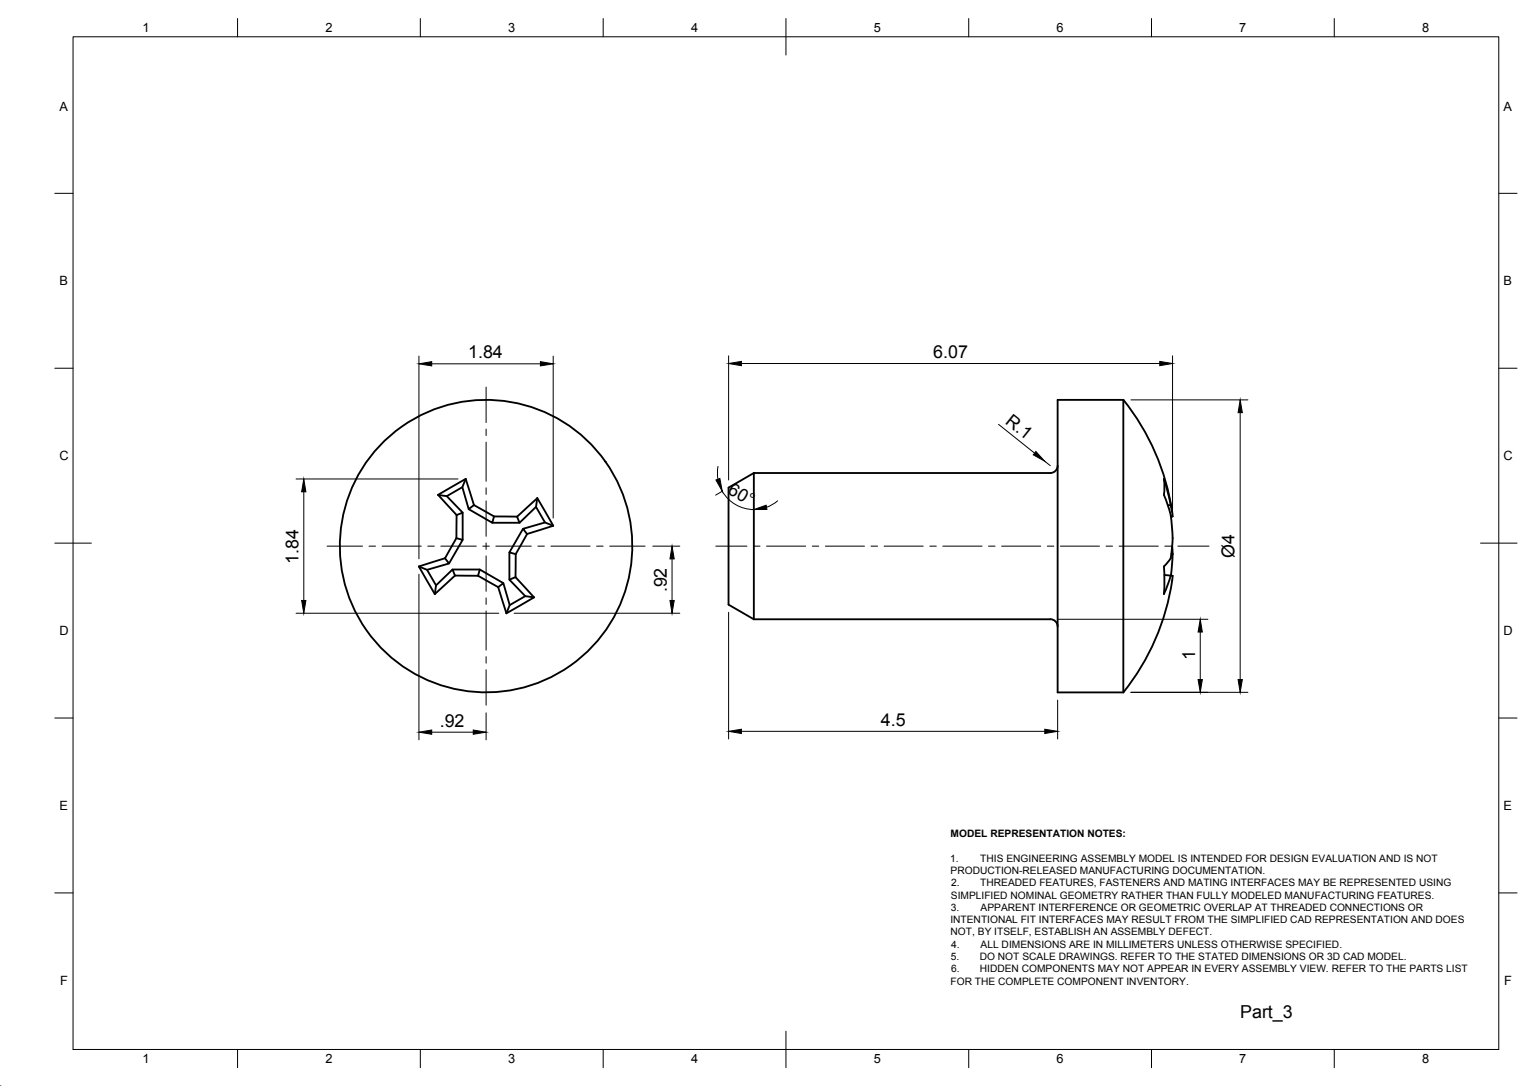
ISO-10303-21;
HEADER;
/* Generated by software containing ST-Developer
 * from STEP Tools, Inc. (www.steptools.com) 
 */

FILE_DESCRIPTION(
/* description */ ('STEP AP242 Edition 2'),
/* implementation_level */ '2;1');

FILE_NAME(
/* name */ 'Part_3.step',
/* time_stamp */ '2026-10-06T10:11:12-07:00',
/* author */ (''),
/* organization */ (''),
/* preprocessor_version */ 'ST-DEVELOPER v20.2',
/* originating_system */ 'Autodesk Translation Framework v15.15.0.0',
/* authorisation */ '');

FILE_SCHEMA (('AUTOMOTIVE_DESIGN { 1 0 10303 214 3 1 1 }'));
ENDSEC;

DATA;
#10=MECHANICAL_DESIGN_GEOMETRIC_PRESENTATION_REPRESENTATION('',(#1796),#54580);
#141=CONICAL_SURFACE('',#19114,0.001,0.5235987755983);
#151=SPHERICAL_SURFACE('',#19080,0.0032);
#260=TOROIDAL_SURFACE('',#19136,0.0011,0.0001);
#1752=SHAPE_REPRESENTATION_RELATIONSHIP('SRR','None',#54639,#1766);
#1766=ADVANCED_BREP_SHAPE_REPRESENTATION('',(#1810),#54575);
#1796=STYLED_ITEM('',(#54716),#1810);
#1810=MANIFOLD_SOLID_BREP('Body1',#17675);
#2262=LINE('',#48636,#2855);
#2263=LINE('',#48644,#2856);
#2264=LINE('',#48647,#2857);
#2265=LINE('',#48650,#2858);
#2266=LINE('',#48652,#2859);
#2267=LINE('',#48653,#2860);
#2268=LINE('',#48656,#2861);
#2269=LINE('',#48657,#2862);
#2270=LINE('',#48660,#2863);
#2271=LINE('',#48661,#2864);
#2272=LINE('',#48664,#2865);
#2273=LINE('',#48665,#2866);
#2274=LINE('',#48668,#2867);
#2275=LINE('',#48669,#2868);
#2276=LINE('',#48672,#2869);
#2277=LINE('',#48673,#2870);
#2278=LINE('',#48676,#2871);
#2279=LINE('',#48677,#2872);
#2280=LINE('',#48680,#2873);
#2281=LINE('',#48681,#2874);
#2282=LINE('',#48684,#2875);
#2283=LINE('',#48685,#2876);
#2284=LINE('',#48688,#2877);
#2285=LINE('',#48689,#2878);
#2286=LINE('',#48692,#2879);
#2287=LINE('',#48693,#2880);
#2288=LINE('',#48696,#2881);
#2289=LINE('',#48697,#2882);
#2290=LINE('',#48700,#2883);
#2291=LINE('',#48701,#2884);
#2292=LINE('',#48704,#2885);
#2293=LINE('',#48705,#2886);
#2294=LINE('',#48708,#2887);
#2295=LINE('',#48709,#2888);
#2296=LINE('',#48712,#2889);
#2297=LINE('',#48713,#2890);
#2298=LINE('',#48716,#2891);
#2299=LINE('',#48717,#2892);
#2300=LINE('',#48720,#2893);
#2301=LINE('',#48721,#2894);
#2302=LINE('',#48724,#2895);
#2303=LINE('',#48725,#2896);
#2304=LINE('',#48727,#2897);
#2855=VECTOR('',#22596,0.002);
#2856=VECTOR('',#22605,0.001);
#2857=VECTOR('',#22610,0.001);
#2858=VECTOR('',#22613,1.);
#2859=VECTOR('',#22614,1.);
#2860=VECTOR('',#22615,1.);
#2861=VECTOR('',#22618,1.);
#2862=VECTOR('',#22619,1.);
#2863=VECTOR('',#22622,1.);
#2864=VECTOR('',#22623,1.);
#2865=VECTOR('',#22626,1.);
#2866=VECTOR('',#22627,1.);
#2867=VECTOR('',#22630,1.);
#2868=VECTOR('',#22631,1.);
#2869=VECTOR('',#22634,0.999999999999999);
#2870=VECTOR('',#22635,1.);
#2871=VECTOR('',#22638,1.);
#2872=VECTOR('',#22639,1.);
#2873=VECTOR('',#22642,1.);
#2874=VECTOR('',#22643,1.);
#2875=VECTOR('',#22646,1.);
#2876=VECTOR('',#22647,1.);
#2877=VECTOR('',#22650,1.);
#2878=VECTOR('',#22651,1.);
#2879=VECTOR('',#22654,1.);
#2880=VECTOR('',#22655,1.);
#2881=VECTOR('',#22658,1.);
#2882=VECTOR('',#22659,1.);
#2883=VECTOR('',#22662,1.);
#2884=VECTOR('',#22663,1.);
#2885=VECTOR('',#22666,1.);
#2886=VECTOR('',#22667,1.);
#2887=VECTOR('',#22670,1.);
#2888=VECTOR('',#22671,1.);
#2889=VECTOR('',#22674,1.);
#2890=VECTOR('',#22675,1.);
#2891=VECTOR('',#22678,1.);
#2892=VECTOR('',#22679,0.999999999999999);
#2893=VECTOR('',#22682,1.);
#2894=VECTOR('',#22683,1.);
#2895=VECTOR('',#22686,1.);
#2896=VECTOR('',#22687,1.);
#2897=VECTOR('',#22690,1.);
#3400=CYLINDRICAL_SURFACE('',#19108,0.002);
#3401=CYLINDRICAL_SURFACE('',#19111,0.001);
#3513=FACE_BOUND('',#5345,.T.);
#4301=FACE_OUTER_BOUND('',#5343,.T.);
#4302=FACE_OUTER_BOUND('',#5344,.T.);
#4303=FACE_OUTER_BOUND('',#5346,.T.);
#4304=FACE_OUTER_BOUND('',#5347,.T.);
#4305=FACE_OUTER_BOUND('',#5348,.T.);
#4306=FACE_OUTER_BOUND('',#5349,.T.);
#4307=FACE_OUTER_BOUND('',#5350,.T.);
#4308=FACE_OUTER_BOUND('',#5351,.T.);
#4309=FACE_OUTER_BOUND('',#5352,.T.);
#4310=FACE_OUTER_BOUND('',#5353,.T.);
#4311=FACE_OUTER_BOUND('',#5354,.T.);
#4312=FACE_OUTER_BOUND('',#5355,.T.);
#4313=FACE_OUTER_BOUND('',#5356,.T.);
#4314=FACE_OUTER_BOUND('',#5357,.T.);
#4315=FACE_OUTER_BOUND('',#5358,.T.);
#4316=FACE_OUTER_BOUND('',#5359,.T.);
#4317=FACE_OUTER_BOUND('',#5360,.T.);
#4318=FACE_OUTER_BOUND('',#5361,.T.);
#4319=FACE_OUTER_BOUND('',#5362,.T.);
#4320=FACE_OUTER_BOUND('',#5363,.T.);
#4321=FACE_OUTER_BOUND('',#5364,.T.);
#4322=FACE_OUTER_BOUND('',#5365,.T.);
#4323=FACE_OUTER_BOUND('',#5366,.T.);
#4324=FACE_OUTER_BOUND('',#5367,.T.);
#4325=FACE_OUTER_BOUND('',#5368,.T.);
#4326=FACE_OUTER_BOUND('',#5369,.T.);
#4327=FACE_OUTER_BOUND('',#5370,.T.);
#4328=FACE_OUTER_BOUND('',#5371,.T.);
#5343=EDGE_LOOP('',(#15325,#15326,#15327,#15328,#15329,#15330,#15331,#15332,
#15333,#15334,#15335,#15336,#15337,#15338,#15339,#15340,#15341,#15342,#15343,
#15344,#15345,#15346,#15347,#15348,#15349));
#5344=EDGE_LOOP('',(#15350));
#5345=EDGE_LOOP('',(#15351));
#5346=EDGE_LOOP('',(#15352,#15353,#15354,#15355,#15356));
#5347=EDGE_LOOP('',(#15357));
#5348=EDGE_LOOP('',(#15358,#15359,#15360,#15361));
#5349=EDGE_LOOP('',(#15362,#15363,#15364,#15365));
#5350=EDGE_LOOP('',(#15366,#15367,#15368,#15369));
#5351=EDGE_LOOP('',(#15370,#15371,#15372,#15373));
#5352=EDGE_LOOP('',(#15374,#15375,#15376,#15377));
#5353=EDGE_LOOP('',(#15378,#15379,#15380,#15381));
#5354=EDGE_LOOP('',(#15382,#15383,#15384,#15385));
#5355=EDGE_LOOP('',(#15386,#15387,#15388,#15389));
#5356=EDGE_LOOP('',(#15390,#15391,#15392,#15393));
#5357=EDGE_LOOP('',(#15394,#15395,#15396,#15397));
#5358=EDGE_LOOP('',(#15398,#15399,#15400,#15401));
#5359=EDGE_LOOP('',(#15402,#15403,#15404,#15405));
#5360=EDGE_LOOP('',(#15406,#15407,#15408,#15409));
#5361=EDGE_LOOP('',(#15410,#15411,#15412,#15413,#15414));
#5362=EDGE_LOOP('',(#15415,#15416,#15417,#15418));
#5363=EDGE_LOOP('',(#15419,#15420,#15421,#15422));
#5364=EDGE_LOOP('',(#15423,#15424,#15425,#15426));
#5365=EDGE_LOOP('',(#15427,#15428,#15429,#15430));
#5366=EDGE_LOOP('',(#15431,#15432,#15433,#15434));
#5367=EDGE_LOOP('',(#15435,#15436,#15437,#15438));
#5368=EDGE_LOOP('',(#15439,#15440,#15441,#15442));
#5369=EDGE_LOOP('',(#15443,#15444,#15445,#15446));
#5370=EDGE_LOOP('',(#15447,#15448,#15449,#15450,#15451,#15452,#15453,#15454,
#15455,#15456,#15457,#15458,#15459,#15460,#15461,#15462,#15463,#15464,#15465,
#15466));
#5371=EDGE_LOOP('',(#15467,#15468,#15469,#15470));
#6242=CIRCLE('',#19081,0.00318247006517847);
#6243=CIRCLE('',#19082,0.00314126219074625);
#6244=CIRCLE('',#19083,0.00318247006517847);
#6245=CIRCLE('',#19084,0.00319919707806175);
#6246=CIRCLE('',#19085,0.00319919707806175);
#6247=CIRCLE('',#19086,0.00318247006517847);
#6248=CIRCLE('',#19087,0.00314126219074625);
#6249=CIRCLE('',#19088,0.00318247006517847);
#6250=CIRCLE('',#19089,0.00319919707806175);
#6251=CIRCLE('',#19090,0.00319919707806175);
#6252=CIRCLE('',#19091,0.00318247006517847);
#6253=CIRCLE('',#19092,0.00314126219074625);
#6254=CIRCLE('',#19093,0.0032);
#6255=CIRCLE('',#19094,0.002);
#6256=CIRCLE('',#19095,0.002);
#6257=CIRCLE('',#19096,0.00314126219074625);
#6258=CIRCLE('',#19097,0.00318247006517847);
#6259=CIRCLE('',#19098,0.00319919707806175);
#6260=CIRCLE('',#19099,0.00319919707806175);
#6261=CIRCLE('',#19100,0.00318247006517847);
#6262=CIRCLE('',#19101,0.00314126219074625);
#6263=CIRCLE('',#19102,0.00318247006517847);
#6264=CIRCLE('',#19103,0.00319919707806175);
#6265=CIRCLE('',#19104,0.00319919707806175);
#6266=CIRCLE('',#19106,0.002);
#6267=CIRCLE('',#19107,0.0011);
#6268=CIRCLE('',#19110,0.0008);
#6269=CIRCLE('',#19112,0.001);
#6270=CIRCLE('',#19113,0.001);
#6271=CIRCLE('',#19137,0.0001);
#7941=VERTEX_POINT('',#48583);
#7942=VERTEX_POINT('',#48584);
#7943=VERTEX_POINT('',#48586);
#7944=VERTEX_POINT('',#48588);
#7945=VERTEX_POINT('',#48590);
#7946=VERTEX_POINT('',#48592);
#7947=VERTEX_POINT('',#48594);
#7948=VERTEX_POINT('',#48596);
#7949=VERTEX_POINT('',#48598);
#7950=VERTEX_POINT('',#48600);
#7951=VERTEX_POINT('',#48602);
#7952=VERTEX_POINT('',#48604);
#7953=VERTEX_POINT('',#48606);
#7954=VERTEX_POINT('',#48608);
#7955=VERTEX_POINT('',#48610);
#7956=VERTEX_POINT('',#48613);
#7957=VERTEX_POINT('',#48615);
#7958=VERTEX_POINT('',#48617);
#7959=VERTEX_POINT('',#48619);
#7960=VERTEX_POINT('',#48621);
#7961=VERTEX_POINT('',#48623);
#7962=VERTEX_POINT('',#48625);
#7963=VERTEX_POINT('',#48627);
#7964=VERTEX_POINT('',#48631);
#7965=VERTEX_POINT('',#48633);
#7966=VERTEX_POINT('',#48638);
#7967=VERTEX_POINT('',#48641);
#7968=VERTEX_POINT('',#48643);
#7969=VERTEX_POINT('',#48649);
#7970=VERTEX_POINT('',#48651);
#7971=VERTEX_POINT('',#48655);
#7972=VERTEX_POINT('',#48659);
#7973=VERTEX_POINT('',#48663);
#7974=VERTEX_POINT('',#48667);
#7975=VERTEX_POINT('',#48671);
#7976=VERTEX_POINT('',#48675);
#7977=VERTEX_POINT('',#48679);
#7978=VERTEX_POINT('',#48683);
#7979=VERTEX_POINT('',#48687);
#7980=VERTEX_POINT('',#48691);
#7981=VERTEX_POINT('',#48695);
#7982=VERTEX_POINT('',#48699);
#7983=VERTEX_POINT('',#48703);
#7984=VERTEX_POINT('',#48707);
#7985=VERTEX_POINT('',#48711);
#7986=VERTEX_POINT('',#48715);
#7987=VERTEX_POINT('',#48719);
#7988=VERTEX_POINT('',#48723);
#10454=EDGE_CURVE('',#7941,#7942,#6242,.F.);
#10455=EDGE_CURVE('',#7943,#7941,#6243,.F.);
#10456=EDGE_CURVE('',#7944,#7943,#6244,.F.);
#10457=EDGE_CURVE('',#7945,#7944,#6245,.F.);
#10458=EDGE_CURVE('',#7946,#7945,#6246,.F.);
#10459=EDGE_CURVE('',#7947,#7946,#6247,.F.);
#10460=EDGE_CURVE('',#7948,#7947,#6248,.F.);
#10461=EDGE_CURVE('',#7949,#7948,#6249,.F.);
#10462=EDGE_CURVE('',#7950,#7949,#6250,.F.);
#10463=EDGE_CURVE('',#7951,#7950,#6251,.F.);
#10464=EDGE_CURVE('',#7952,#7951,#6252,.F.);
#10465=EDGE_CURVE('',#7953,#7952,#6253,.F.);
#10466=EDGE_CURVE('',#7953,#7954,#6254,.T.);
#10467=EDGE_CURVE('',#7954,#7955,#6255,.T.);
#10468=EDGE_CURVE('',#7955,#7954,#6256,.T.);
#10469=EDGE_CURVE('',#7956,#7953,#6257,.F.);
#10470=EDGE_CURVE('',#7957,#7956,#6258,.F.);
#10471=EDGE_CURVE('',#7958,#7957,#6259,.F.);
#10472=EDGE_CURVE('',#7959,#7958,#6260,.F.);
#10473=EDGE_CURVE('',#7960,#7959,#6261,.F.);
#10474=EDGE_CURVE('',#7961,#7960,#6262,.F.);
#10475=EDGE_CURVE('',#7962,#7961,#6263,.F.);
#10476=EDGE_CURVE('',#7963,#7962,#6264,.F.);
#10477=EDGE_CURVE('',#7942,#7963,#6265,.F.);
#10478=EDGE_CURVE('',#7964,#7964,#6266,.T.);
#10479=EDGE_CURVE('',#7965,#7965,#6267,.T.);
#10480=EDGE_CURVE('',#7955,#7964,#2262,.T.);
#10481=EDGE_CURVE('',#7966,#7966,#6268,.F.);
#10482=EDGE_CURVE('',#7967,#7967,#6269,.F.);
#10483=EDGE_CURVE('',#7967,#7968,#2263,.T.);
#10484=EDGE_CURVE('',#7968,#7968,#6270,.T.);
#10485=EDGE_CURVE('',#7968,#7966,#2264,.T.);
#10486=EDGE_CURVE('',#7969,#7942,#2265,.T.);
#10487=EDGE_CURVE('',#7969,#7970,#2266,.F.);
#10488=EDGE_CURVE('',#7970,#7941,#2267,.T.);
#10489=EDGE_CURVE('',#7970,#7971,#2268,.F.);
#10490=EDGE_CURVE('',#7971,#7943,#2269,.T.);
#10491=EDGE_CURVE('',#7971,#7972,#2270,.F.);
#10492=EDGE_CURVE('',#7972,#7944,#2271,.T.);
#10493=EDGE_CURVE('',#7972,#7973,#2272,.F.);
#10494=EDGE_CURVE('',#7973,#7945,#2273,.T.);
#10495=EDGE_CURVE('',#7973,#7974,#2274,.F.);
#10496=EDGE_CURVE('',#7974,#7946,#2275,.T.);
#10497=EDGE_CURVE('',#7974,#7975,#2276,.F.);
#10498=EDGE_CURVE('',#7975,#7947,#2277,.T.);
#10499=EDGE_CURVE('',#7975,#7976,#2278,.F.);
#10500=EDGE_CURVE('',#7976,#7948,#2279,.T.);
#10501=EDGE_CURVE('',#7976,#7977,#2280,.F.);
#10502=EDGE_CURVE('',#7977,#7949,#2281,.T.);
#10503=EDGE_CURVE('',#7977,#7978,#2282,.F.);
#10504=EDGE_CURVE('',#7978,#7950,#2283,.T.);
#10505=EDGE_CURVE('',#7978,#7979,#2284,.F.);
#10506=EDGE_CURVE('',#7979,#7951,#2285,.T.);
#10507=EDGE_CURVE('',#7979,#7980,#2286,.F.);
#10508=EDGE_CURVE('',#7980,#7952,#2287,.T.);
#10509=EDGE_CURVE('',#7980,#7981,#2288,.F.);
#10510=EDGE_CURVE('',#7981,#7956,#2289,.T.);
#10511=EDGE_CURVE('',#7981,#7982,#2290,.F.);
#10512=EDGE_CURVE('',#7982,#7957,#2291,.T.);
#10513=EDGE_CURVE('',#7982,#7983,#2292,.F.);
#10514=EDGE_CURVE('',#7983,#7958,#2293,.T.);
#10515=EDGE_CURVE('',#7983,#7984,#2294,.F.);
#10516=EDGE_CURVE('',#7984,#7959,#2295,.T.);
#10517=EDGE_CURVE('',#7984,#7985,#2296,.F.);
#10518=EDGE_CURVE('',#7985,#7960,#2297,.T.);
#10519=EDGE_CURVE('',#7985,#7986,#2298,.F.);
#10520=EDGE_CURVE('',#7986,#7961,#2299,.T.);
#10521=EDGE_CURVE('',#7986,#7987,#2300,.F.);
#10522=EDGE_CURVE('',#7987,#7962,#2301,.T.);
#10523=EDGE_CURVE('',#7987,#7988,#2302,.F.);
#10524=EDGE_CURVE('',#7988,#7963,#2303,.T.);
#10525=EDGE_CURVE('',#7988,#7969,#2304,.F.);
#10526=EDGE_CURVE('',#7965,#7967,#6271,.T.);
#15325=ORIENTED_EDGE('',*,*,#10454,.F.);
#15326=ORIENTED_EDGE('',*,*,#10455,.F.);
#15327=ORIENTED_EDGE('',*,*,#10456,.F.);
#15328=ORIENTED_EDGE('',*,*,#10457,.F.);
#15329=ORIENTED_EDGE('',*,*,#10458,.F.);
#15330=ORIENTED_EDGE('',*,*,#10459,.F.);
#15331=ORIENTED_EDGE('',*,*,#10460,.F.);
#15332=ORIENTED_EDGE('',*,*,#10461,.F.);
#15333=ORIENTED_EDGE('',*,*,#10462,.F.);
#15334=ORIENTED_EDGE('',*,*,#10463,.F.);
#15335=ORIENTED_EDGE('',*,*,#10464,.F.);
#15336=ORIENTED_EDGE('',*,*,#10465,.F.);
#15337=ORIENTED_EDGE('',*,*,#10466,.T.);
#15338=ORIENTED_EDGE('',*,*,#10467,.T.);
#15339=ORIENTED_EDGE('',*,*,#10468,.T.);
#15340=ORIENTED_EDGE('',*,*,#10466,.F.);
#15341=ORIENTED_EDGE('',*,*,#10469,.F.);
#15342=ORIENTED_EDGE('',*,*,#10470,.F.);
#15343=ORIENTED_EDGE('',*,*,#10471,.F.);
#15344=ORIENTED_EDGE('',*,*,#10472,.F.);
#15345=ORIENTED_EDGE('',*,*,#10473,.F.);
#15346=ORIENTED_EDGE('',*,*,#10474,.F.);
#15347=ORIENTED_EDGE('',*,*,#10475,.F.);
#15348=ORIENTED_EDGE('',*,*,#10476,.F.);
#15349=ORIENTED_EDGE('',*,*,#10477,.F.);
#15350=ORIENTED_EDGE('',*,*,#10478,.F.);
#15351=ORIENTED_EDGE('',*,*,#10479,.T.);
#15352=ORIENTED_EDGE('',*,*,#10467,.F.);
#15353=ORIENTED_EDGE('',*,*,#10468,.F.);
#15354=ORIENTED_EDGE('',*,*,#10480,.T.);
#15355=ORIENTED_EDGE('',*,*,#10478,.T.);
#15356=ORIENTED_EDGE('',*,*,#10480,.F.);
#15357=ORIENTED_EDGE('',*,*,#10481,.T.);
#15358=ORIENTED_EDGE('',*,*,#10482,.T.);
#15359=ORIENTED_EDGE('',*,*,#10483,.T.);
#15360=ORIENTED_EDGE('',*,*,#10484,.T.);
#15361=ORIENTED_EDGE('',*,*,#10483,.F.);
#15362=ORIENTED_EDGE('',*,*,#10484,.F.);
#15363=ORIENTED_EDGE('',*,*,#10485,.T.);
#15364=ORIENTED_EDGE('',*,*,#10481,.F.);
#15365=ORIENTED_EDGE('',*,*,#10485,.F.);
#15366=ORIENTED_EDGE('',*,*,#10454,.T.);
#15367=ORIENTED_EDGE('',*,*,#10486,.F.);
#15368=ORIENTED_EDGE('',*,*,#10487,.T.);
#15369=ORIENTED_EDGE('',*,*,#10488,.T.);
#15370=ORIENTED_EDGE('',*,*,#10455,.T.);
#15371=ORIENTED_EDGE('',*,*,#10488,.F.);
#15372=ORIENTED_EDGE('',*,*,#10489,.T.);
#15373=ORIENTED_EDGE('',*,*,#10490,.T.);
#15374=ORIENTED_EDGE('',*,*,#10456,.T.);
#15375=ORIENTED_EDGE('',*,*,#10490,.F.);
#15376=ORIENTED_EDGE('',*,*,#10491,.T.);
#15377=ORIENTED_EDGE('',*,*,#10492,.T.);
#15378=ORIENTED_EDGE('',*,*,#10457,.T.);
#15379=ORIENTED_EDGE('',*,*,#10492,.F.);
#15380=ORIENTED_EDGE('',*,*,#10493,.T.);
#15381=ORIENTED_EDGE('',*,*,#10494,.T.);
#15382=ORIENTED_EDGE('',*,*,#10458,.T.);
#15383=ORIENTED_EDGE('',*,*,#10494,.F.);
#15384=ORIENTED_EDGE('',*,*,#10495,.T.);
#15385=ORIENTED_EDGE('',*,*,#10496,.T.);
#15386=ORIENTED_EDGE('',*,*,#10459,.T.);
#15387=ORIENTED_EDGE('',*,*,#10496,.F.);
#15388=ORIENTED_EDGE('',*,*,#10497,.T.);
#15389=ORIENTED_EDGE('',*,*,#10498,.T.);
#15390=ORIENTED_EDGE('',*,*,#10460,.T.);
#15391=ORIENTED_EDGE('',*,*,#10498,.F.);
#15392=ORIENTED_EDGE('',*,*,#10499,.T.);
#15393=ORIENTED_EDGE('',*,*,#10500,.T.);
#15394=ORIENTED_EDGE('',*,*,#10461,.T.);
#15395=ORIENTED_EDGE('',*,*,#10500,.F.);
#15396=ORIENTED_EDGE('',*,*,#10501,.T.);
#15397=ORIENTED_EDGE('',*,*,#10502,.T.);
#15398=ORIENTED_EDGE('',*,*,#10462,.T.);
#15399=ORIENTED_EDGE('',*,*,#10502,.F.);
#15400=ORIENTED_EDGE('',*,*,#10503,.T.);
#15401=ORIENTED_EDGE('',*,*,#10504,.T.);
#15402=ORIENTED_EDGE('',*,*,#10463,.T.);
#15403=ORIENTED_EDGE('',*,*,#10504,.F.);
#15404=ORIENTED_EDGE('',*,*,#10505,.T.);
#15405=ORIENTED_EDGE('',*,*,#10506,.T.);
#15406=ORIENTED_EDGE('',*,*,#10464,.T.);
#15407=ORIENTED_EDGE('',*,*,#10506,.F.);
#15408=ORIENTED_EDGE('',*,*,#10507,.T.);
#15409=ORIENTED_EDGE('',*,*,#10508,.T.);
#15410=ORIENTED_EDGE('',*,*,#10469,.T.);
#15411=ORIENTED_EDGE('',*,*,#10465,.T.);
#15412=ORIENTED_EDGE('',*,*,#10508,.F.);
#15413=ORIENTED_EDGE('',*,*,#10509,.T.);
#15414=ORIENTED_EDGE('',*,*,#10510,.T.);
#15415=ORIENTED_EDGE('',*,*,#10470,.T.);
#15416=ORIENTED_EDGE('',*,*,#10510,.F.);
#15417=ORIENTED_EDGE('',*,*,#10511,.T.);
#15418=ORIENTED_EDGE('',*,*,#10512,.T.);
#15419=ORIENTED_EDGE('',*,*,#10471,.T.);
#15420=ORIENTED_EDGE('',*,*,#10512,.F.);
#15421=ORIENTED_EDGE('',*,*,#10513,.T.);
#15422=ORIENTED_EDGE('',*,*,#10514,.T.);
#15423=ORIENTED_EDGE('',*,*,#10472,.T.);
#15424=ORIENTED_EDGE('',*,*,#10514,.F.);
#15425=ORIENTED_EDGE('',*,*,#10515,.T.);
#15426=ORIENTED_EDGE('',*,*,#10516,.T.);
#15427=ORIENTED_EDGE('',*,*,#10473,.T.);
#15428=ORIENTED_EDGE('',*,*,#10516,.F.);
#15429=ORIENTED_EDGE('',*,*,#10517,.T.);
#15430=ORIENTED_EDGE('',*,*,#10518,.T.);
#15431=ORIENTED_EDGE('',*,*,#10474,.T.);
#15432=ORIENTED_EDGE('',*,*,#10518,.F.);
#15433=ORIENTED_EDGE('',*,*,#10519,.T.);
#15434=ORIENTED_EDGE('',*,*,#10520,.T.);
#15435=ORIENTED_EDGE('',*,*,#10475,.T.);
#15436=ORIENTED_EDGE('',*,*,#10520,.F.);
#15437=ORIENTED_EDGE('',*,*,#10521,.T.);
#15438=ORIENTED_EDGE('',*,*,#10522,.T.);
#15439=ORIENTED_EDGE('',*,*,#10476,.T.);
#15440=ORIENTED_EDGE('',*,*,#10522,.F.);
#15441=ORIENTED_EDGE('',*,*,#10523,.T.);
#15442=ORIENTED_EDGE('',*,*,#10524,.T.);
#15443=ORIENTED_EDGE('',*,*,#10477,.T.);
#15444=ORIENTED_EDGE('',*,*,#10524,.F.);
#15445=ORIENTED_EDGE('',*,*,#10525,.T.);
#15446=ORIENTED_EDGE('',*,*,#10486,.T.);
#15447=ORIENTED_EDGE('',*,*,#10487,.F.);
#15448=ORIENTED_EDGE('',*,*,#10525,.F.);
#15449=ORIENTED_EDGE('',*,*,#10523,.F.);
#15450=ORIENTED_EDGE('',*,*,#10521,.F.);
#15451=ORIENTED_EDGE('',*,*,#10519,.F.);
#15452=ORIENTED_EDGE('',*,*,#10517,.F.);
#15453=ORIENTED_EDGE('',*,*,#10515,.F.);
#15454=ORIENTED_EDGE('',*,*,#10513,.F.);
#15455=ORIENTED_EDGE('',*,*,#10511,.F.);
#15456=ORIENTED_EDGE('',*,*,#10509,.F.);
#15457=ORIENTED_EDGE('',*,*,#10507,.F.);
#15458=ORIENTED_EDGE('',*,*,#10505,.F.);
#15459=ORIENTED_EDGE('',*,*,#10503,.F.);
#15460=ORIENTED_EDGE('',*,*,#10501,.F.);
#15461=ORIENTED_EDGE('',*,*,#10499,.F.);
#15462=ORIENTED_EDGE('',*,*,#10497,.F.);
#15463=ORIENTED_EDGE('',*,*,#10495,.F.);
#15464=ORIENTED_EDGE('',*,*,#10493,.F.);
#15465=ORIENTED_EDGE('',*,*,#10491,.F.);
#15466=ORIENTED_EDGE('',*,*,#10489,.F.);
#15467=ORIENTED_EDGE('',*,*,#10479,.F.);
#15468=ORIENTED_EDGE('',*,*,#10526,.T.);
#15469=ORIENTED_EDGE('',*,*,#10482,.F.);
#15470=ORIENTED_EDGE('',*,*,#10526,.F.);
#16614=PLANE('',#19105);
#16615=PLANE('',#19109);
#16616=PLANE('',#19115);
#16617=PLANE('',#19116);
#16618=PLANE('',#19117);
#16619=PLANE('',#19118);
#16620=PLANE('',#19119);
#16621=PLANE('',#19120);
#16622=PLANE('',#19121);
#16623=PLANE('',#19122);
#16624=PLANE('',#19123);
#16625=PLANE('',#19124);
#16626=PLANE('',#19125);
#16627=PLANE('',#19126);
#16628=PLANE('',#19127);
#16629=PLANE('',#19128);
#16630=PLANE('',#19129);
#16631=PLANE('',#19130);
#16632=PLANE('',#19131);
#16633=PLANE('',#19132);
#16634=PLANE('',#19133);
#16635=PLANE('',#19134);
#16636=PLANE('',#19135);
#17417=ADVANCED_FACE('',(#4301),#151,.T.);
#17418=ADVANCED_FACE('',(#4302,#3513),#16614,.F.);
#17419=ADVANCED_FACE('',(#4303),#3400,.T.);
#17420=ADVANCED_FACE('',(#4304),#16615,.F.);
#17421=ADVANCED_FACE('',(#4305),#3401,.T.);
#17422=ADVANCED_FACE('',(#4306),#141,.T.);
#17423=ADVANCED_FACE('',(#4307),#16616,.F.);
#17424=ADVANCED_FACE('',(#4308),#16617,.F.);
#17425=ADVANCED_FACE('',(#4309),#16618,.F.);
#17426=ADVANCED_FACE('',(#4310),#16619,.F.);
#17427=ADVANCED_FACE('',(#4311),#16620,.F.);
#17428=ADVANCED_FACE('',(#4312),#16621,.F.);
#17429=ADVANCED_FACE('',(#4313),#16622,.F.);
#17430=ADVANCED_FACE('',(#4314),#16623,.F.);
#17431=ADVANCED_FACE('',(#4315),#16624,.F.);
#17432=ADVANCED_FACE('',(#4316),#16625,.F.);
#17433=ADVANCED_FACE('',(#4317),#16626,.F.);
#17434=ADVANCED_FACE('',(#4318),#16627,.F.);
#17435=ADVANCED_FACE('',(#4319),#16628,.F.);
#17436=ADVANCED_FACE('',(#4320),#16629,.F.);
#17437=ADVANCED_FACE('',(#4321),#16630,.F.);
#17438=ADVANCED_FACE('',(#4322),#16631,.F.);
#17439=ADVANCED_FACE('',(#4323),#16632,.F.);
#17440=ADVANCED_FACE('',(#4324),#16633,.F.);
#17441=ADVANCED_FACE('',(#4325),#16634,.F.);
#17442=ADVANCED_FACE('',(#4326),#16635,.F.);
#17443=ADVANCED_FACE('',(#4327),#16636,.T.);
#17444=ADVANCED_FACE('',(#4328),#260,.F.);
#17675=CLOSED_SHELL('',(#17417,#17418,#17419,#17420,#17421,#17422,#17423,
#17424,#17425,#17426,#17427,#17428,#17429,#17430,#17431,#17432,#17433,#17434,
#17435,#17436,#17437,#17438,#17439,#17440,#17441,#17442,#17443,#17444));
#19079=AXIS2_PLACEMENT_3D('',#48581,#22536,#22537);
#19080=AXIS2_PLACEMENT_3D('',#48582,#22538,#22539);
#19081=AXIS2_PLACEMENT_3D('',#48585,#22540,#22541);
#19082=AXIS2_PLACEMENT_3D('',#48587,#22542,#22543);
#19083=AXIS2_PLACEMENT_3D('',#48589,#22544,#22545);
#19084=AXIS2_PLACEMENT_3D('',#48591,#22546,#22547);
#19085=AXIS2_PLACEMENT_3D('',#48593,#22548,#22549);
#19086=AXIS2_PLACEMENT_3D('',#48595,#22550,#22551);
#19087=AXIS2_PLACEMENT_3D('',#48597,#22552,#22553);
#19088=AXIS2_PLACEMENT_3D('',#48599,#22554,#22555);
#19089=AXIS2_PLACEMENT_3D('',#48601,#22556,#22557);
#19090=AXIS2_PLACEMENT_3D('',#48603,#22558,#22559);
#19091=AXIS2_PLACEMENT_3D('',#48605,#22560,#22561);
#19092=AXIS2_PLACEMENT_3D('',#48607,#22562,#22563);
#19093=AXIS2_PLACEMENT_3D('',#48609,#22564,#22565);
#19094=AXIS2_PLACEMENT_3D('',#48611,#22566,#22567);
#19095=AXIS2_PLACEMENT_3D('',#48612,#22568,#22569);
#19096=AXIS2_PLACEMENT_3D('',#48614,#22570,#22571);
#19097=AXIS2_PLACEMENT_3D('',#48616,#22572,#22573);
#19098=AXIS2_PLACEMENT_3D('',#48618,#22574,#22575);
#19099=AXIS2_PLACEMENT_3D('',#48620,#22576,#22577);
#19100=AXIS2_PLACEMENT_3D('',#48622,#22578,#22579);
#19101=AXIS2_PLACEMENT_3D('',#48624,#22580,#22581);
#19102=AXIS2_PLACEMENT_3D('',#48626,#22582,#22583);
#19103=AXIS2_PLACEMENT_3D('',#48628,#22584,#22585);
#19104=AXIS2_PLACEMENT_3D('',#48629,#22586,#22587);
#19105=AXIS2_PLACEMENT_3D('',#48630,#22588,#22589);
#19106=AXIS2_PLACEMENT_3D('',#48632,#22590,#22591);
#19107=AXIS2_PLACEMENT_3D('',#48634,#22592,#22593);
#19108=AXIS2_PLACEMENT_3D('',#48635,#22594,#22595);
#19109=AXIS2_PLACEMENT_3D('',#48637,#22597,#22598);
#19110=AXIS2_PLACEMENT_3D('',#48639,#22599,#22600);
#19111=AXIS2_PLACEMENT_3D('',#48640,#22601,#22602);
#19112=AXIS2_PLACEMENT_3D('',#48642,#22603,#22604);
#19113=AXIS2_PLACEMENT_3D('',#48645,#22606,#22607);
#19114=AXIS2_PLACEMENT_3D('',#48646,#22608,#22609);
#19115=AXIS2_PLACEMENT_3D('',#48648,#22611,#22612);
#19116=AXIS2_PLACEMENT_3D('',#48654,#22616,#22617);
#19117=AXIS2_PLACEMENT_3D('',#48658,#22620,#22621);
#19118=AXIS2_PLACEMENT_3D('',#48662,#22624,#22625);
#19119=AXIS2_PLACEMENT_3D('',#48666,#22628,#22629);
#19120=AXIS2_PLACEMENT_3D('',#48670,#22632,#22633);
#19121=AXIS2_PLACEMENT_3D('',#48674,#22636,#22637);
#19122=AXIS2_PLACEMENT_3D('',#48678,#22640,#22641);
#19123=AXIS2_PLACEMENT_3D('',#48682,#22644,#22645);
#19124=AXIS2_PLACEMENT_3D('',#48686,#22648,#22649);
#19125=AXIS2_PLACEMENT_3D('',#48690,#22652,#22653);
#19126=AXIS2_PLACEMENT_3D('',#48694,#22656,#22657);
#19127=AXIS2_PLACEMENT_3D('',#48698,#22660,#22661);
#19128=AXIS2_PLACEMENT_3D('',#48702,#22664,#22665);
#19129=AXIS2_PLACEMENT_3D('',#48706,#22668,#22669);
#19130=AXIS2_PLACEMENT_3D('',#48710,#22672,#22673);
#19131=AXIS2_PLACEMENT_3D('',#48714,#22676,#22677);
#19132=AXIS2_PLACEMENT_3D('',#48718,#22680,#22681);
#19133=AXIS2_PLACEMENT_3D('',#48722,#22684,#22685);
#19134=AXIS2_PLACEMENT_3D('',#48726,#22688,#22689);
#19135=AXIS2_PLACEMENT_3D('',#48728,#22691,#22692);
#19136=AXIS2_PLACEMENT_3D('',#48729,#22693,#22694);
#19137=AXIS2_PLACEMENT_3D('',#48730,#22695,#22696);
#22536=DIRECTION('axis',(0.,0.,1.));
#22537=DIRECTION('refdir',(1.,0.,0.));
#22538=DIRECTION('center_axis',(-1.,6.12323399573677E-17,0.));
#22539=DIRECTION('ref_axis',(0.,1.,0.));
#22540=DIRECTION('center_axis',(0.104528463267654,-0.241206989505463,-0.964827958021851));
#22541=DIRECTION('ref_axis',(1.25352732846412E-16,0.970142500145332,-0.242535625036333));
#22542=DIRECTION('center_axis',(0.104528463267654,0.994521895368273,0.));
#22543=DIRECTION('ref_axis',(-0.994521895368273,0.104528463267654,0.));
#22544=DIRECTION('center_axis',(0.104528463267654,-0.241206989505463,0.964827958021851));
#22545=DIRECTION('ref_axis',(-1.25352732846412E-16,-0.970142500145332,-0.242535625036333));
#22546=DIRECTION('center_axis',(0.104528463267654,0.497260947684128,0.861281226008779));
#22547=DIRECTION('ref_axis',(-4.48880618532109E-17,-0.866025403784444,0.499999999999991));
#22548=DIRECTION('center_axis',(0.104528463267654,0.861281226008788,0.497260947684113));
#22549=DIRECTION('ref_axis',(4.7859022490904E-17,-0.499999999999977,0.866025403784452));
#22550=DIRECTION('center_axis',(0.104528463267654,0.964827958021848,-0.241206989505473));
#22551=DIRECTION('ref_axis',(3.35494973080118E-17,0.242535625036343,0.970142500145329));
#22552=DIRECTION('center_axis',(0.104528463267654,1.0442123953466E-14,0.994521895368273));
#22553=DIRECTION('ref_axis',(0.994521895368273,2.35340993718907E-32,-0.104528463267654));
#22554=DIRECTION('center_axis',(0.104528463267654,-0.964827958021853,-0.241206989505453));
#22555=DIRECTION('ref_axis',(-1.87869149990428E-17,0.242535625036323,-0.970142500145334));
#22556=DIRECTION('center_axis',(0.104528463267654,-0.861281226008775,0.497260947684136));
#22557=DIRECTION('ref_axis',(-8.84532624015479E-17,-0.499999999999999,-0.866025403784439));
#22558=DIRECTION('center_axis',(0.104528463267654,-0.497260947684123,0.861281226008782));
#22559=DIRECTION('ref_axis',(-4.87589202125001E-17,-0.866025403784447,-0.499999999999986));
#22560=DIRECTION('center_axis',(0.104528463267654,0.241206989505469,0.964827958021849));
#22561=DIRECTION('ref_axis',(3.21756749545783E-17,-0.97014250014533,0.242535625036339));
#22562=DIRECTION('center_axis',(0.104528463267654,-0.994521895368273,6.81008083921694E-15));
#22563=DIRECTION('ref_axis',(0.994521895368273,0.104528463267654,-2.74588614067193E-32));
#22564=DIRECTION('center_axis',(0.,1.22464679914735E-16,1.));
#22565=DIRECTION('ref_axis',(0.,-1.,1.22464679914735E-16));
#22566=DIRECTION('center_axis',(-1.,0.,0.));
#22567=DIRECTION('ref_axis',(0.,0.,1.));
#22568=DIRECTION('center_axis',(-1.,0.,0.));
#22569=DIRECTION('ref_axis',(0.,0.,1.));
#22570=DIRECTION('center_axis',(0.104528463267654,-0.994521895368273,6.81008083921694E-15));
#22571=DIRECTION('ref_axis',(0.994521895368273,0.104528463267654,-2.74588614067193E-32));
#22572=DIRECTION('center_axis',(0.104528463267654,0.241206989505456,-0.964827958021853));
#22573=DIRECTION('ref_axis',(-2.00678541197572E-17,0.970142500145334,0.242535625036326));
#22574=DIRECTION('center_axis',(0.104528463267654,-0.497260947684145,-0.861281226008769));
#22575=DIRECTION('ref_axis',(-1.75746881493118E-17,0.866025403784434,-0.500000000000009));
#22576=DIRECTION('center_axis',(0.104528463267654,-0.861281226008775,-0.497260947684136));
#22577=DIRECTION('ref_axis',(8.84532624015479E-17,0.499999999999999,-0.866025403784439));
#22578=DIRECTION('center_axis',(0.104528463267654,-0.96482795802185,0.241206989505466));
#22579=DIRECTION('ref_axis',(3.16327731693601E-17,-0.242535625036336,-0.970142500145331));
#22580=DIRECTION('center_axis',(0.104528463267654,-3.63204311424904E-15,
-0.994521895368273));
#22581=DIRECTION('ref_axis',(-0.994521895368273,-6.31025267670437E-32,-0.104528463267654));
#22582=DIRECTION('center_axis',(0.104528463267654,0.964827958021852,0.241206989505459));
#22583=DIRECTION('ref_axis',(-2.43308567694987E-17,-0.242535625036329,0.970142500145333));
#22584=DIRECTION('center_axis',(0.104528463267654,0.861281226008778,-0.49726094768413));
#22585=DIRECTION('ref_axis',(5.38148870333637E-17,0.499999999999993,0.866025403784443));
#22586=DIRECTION('center_axis',(0.104528463267654,0.497260947684129,-0.861281226008779));
#22587=DIRECTION('ref_axis',(2.61266480593264E-18,0.866025403784443,0.499999999999992));
#22588=DIRECTION('center_axis',(-1.,0.,0.));
#22589=DIRECTION('ref_axis',(0.,0.,1.));
#22590=DIRECTION('center_axis',(-1.,0.,0.));
#22591=DIRECTION('ref_axis',(0.,0.,1.));
#22592=DIRECTION('center_axis',(-1.,0.,0.));
#22593=DIRECTION('ref_axis',(0.,0.,1.));
#22594=DIRECTION('center_axis',(-1.,0.,0.));
#22595=DIRECTION('ref_axis',(0.,0.,1.));
#22596=DIRECTION('',(1.,0.,0.));
#22597=DIRECTION('center_axis',(-1.,0.,0.));
#22598=DIRECTION('ref_axis',(0.,0.,1.));
#22599=DIRECTION('center_axis',(-1.,0.,0.));
#22600=DIRECTION('ref_axis',(0.,0.,1.));
#22601=DIRECTION('center_axis',(-1.,0.,0.));
#22602=DIRECTION('ref_axis',(0.,0.,1.));
#22603=DIRECTION('center_axis',(-1.,0.,0.));
#22604=DIRECTION('ref_axis',(0.,0.,1.));
#22605=DIRECTION('',(1.,0.,0.));
#22606=DIRECTION('center_axis',(-1.,0.,0.));
#22607=DIRECTION('ref_axis',(0.,0.,1.));
#22608=DIRECTION('center_axis',(-1.,0.,0.));
#22609=DIRECTION('ref_axis',(0.,0.,1.));
#22610=DIRECTION('',(0.866025403784438,6.12323399573678E-17,0.500000000000001));
#22611=DIRECTION('center_axis',(0.104528463267654,-0.241206989505463,-0.964827958021851));
#22612=DIRECTION('ref_axis',(1.25352732846412E-16,0.970142500145332,-0.242535625036333));
#22613=DIRECTION('',(-0.993634572314886,0.0156427600493605,-0.111560032084303));
#22614=DIRECTION('',(0.,-0.970142500145332,0.242535625036332));
#22615=DIRECTION('',(-0.985727427293419,0.103604127426078,-0.132693722013437));
#22616=DIRECTION('center_axis',(0.104528463267654,0.994521895368273,0.));
#22617=DIRECTION('ref_axis',(-0.994521895368273,0.104528463267654,0.));
#22618=DIRECTION('',(0.,0.,-1.));
#22619=DIRECTION('',(-0.985727427293419,0.103604127426078,0.132693722013437));
#22620=DIRECTION('center_axis',(0.104528463267654,-0.241206989505463,0.964827958021851));
#22621=DIRECTION('ref_axis',(-1.25352732846412E-16,-0.970142500145332,-0.242535625036333));
#22622=DIRECTION('',(0.,0.970142500145332,0.242535625036332));
#22623=DIRECTION('',(-0.993634572314886,0.0156427600493605,0.111560032084303));
#22624=DIRECTION('center_axis',(0.104528463267654,0.497260947684128,0.861281226008779));
#22625=DIRECTION('ref_axis',(-4.48880618532109E-17,-0.866025403784444,0.499999999999991));
#22626=DIRECTION('',(0.,0.866025403784443,-0.499999999999992));
#22627=DIRECTION('',(-0.994132040497618,0.0764901498757915,0.0764901498757902));
#22628=DIRECTION('center_axis',(0.104528463267654,0.861281226008788,0.497260947684113));
#22629=DIRECTION('ref_axis',(4.7859022490904E-17,-0.499999999999977,0.866025403784452));
#22630=DIRECTION('',(0.,0.499999999999977,-0.866025403784452));
#22631=DIRECTION('',(-0.993634572314886,0.111560032084303,0.0156427600493589));
#22632=DIRECTION('center_axis',(0.104528463267654,0.964827958021848,-0.241206989505473));
#22633=DIRECTION('ref_axis',(3.35494973080118E-17,0.242535625036343,0.970142500145329));
#22634=DIRECTION('',(0.,-0.242535625036343,-0.970142500145329));
#22635=DIRECTION('',(-0.985727427293419,0.132693722013438,0.103604127426076));
#22636=DIRECTION('center_axis',(0.104528463267654,1.0442123953466E-14,0.994521895368273));
#22637=DIRECTION('ref_axis',(0.994521895368273,2.35340993718907E-32,-0.104528463267654));
#22638=DIRECTION('',(0.,1.,-1.04996420914386E-14));
#22639=DIRECTION('',(-0.985727427293419,-0.132693722013436,0.103604127426079));
#22640=DIRECTION('center_axis',(0.104528463267654,-0.964827958021853,-0.241206989505453));
#22641=DIRECTION('ref_axis',(-1.87869149990428E-17,0.242535625036323,-0.970142500145334));
#22642=DIRECTION('',(0.,-0.242535625036323,0.970142500145334));
#22643=DIRECTION('',(-0.993634572314887,-0.111560032084302,0.0156427600493615));
#22644=DIRECTION('center_axis',(0.104528463267654,-0.861281226008775,0.497260947684136));
#22645=DIRECTION('ref_axis',(-8.84532624015479E-17,-0.499999999999999,-0.866025403784439));
#22646=DIRECTION('',(0.,0.5,0.866025403784439));
#22647=DIRECTION('',(-0.994132040497618,-0.07649014987579,0.0764901498757912));
#22648=DIRECTION('center_axis',(0.104528463267654,-0.497260947684123,0.861281226008782));
#22649=DIRECTION('ref_axis',(-4.87589202125001E-17,-0.866025403784447,-0.499999999999986));
#22650=DIRECTION('',(0.,0.866025403784447,0.499999999999986));
#22651=DIRECTION('',(-0.993634572314886,-0.0156427600493598,0.111560032084303));
#22652=DIRECTION('center_axis',(0.104528463267654,0.241206989505469,0.964827958021849));
#22653=DIRECTION('ref_axis',(3.21756749545783E-17,-0.97014250014533,0.242535625036339));
#22654=DIRECTION('',(0.,0.97014250014533,-0.242535625036339));
#22655=DIRECTION('',(-0.985727427293419,-0.103604127426077,0.132693722013437));
#22656=DIRECTION('center_axis',(0.104528463267654,-0.994521895368273,6.81008083921694E-15));
#22657=DIRECTION('ref_axis',(0.994521895368273,0.104528463267654,-2.74588614067193E-32));
#22658=DIRECTION('',(0.,6.8475926683295E-15,1.));
#22659=DIRECTION('',(-0.985727427293419,-0.103604127426079,-0.132693722013436));
#22660=DIRECTION('center_axis',(0.104528463267654,0.241206989505456,-0.964827958021853));
#22661=DIRECTION('ref_axis',(-2.00678541197572E-17,0.970142500145334,0.242535625036326));
#22662=DIRECTION('',(0.,-0.970142500145334,-0.242535625036326));
#22663=DIRECTION('',(-0.993634572314886,-0.015642760049362,-0.111560032084303));
#22664=DIRECTION('center_axis',(0.104528463267654,-0.497260947684145,-0.861281226008769));
#22665=DIRECTION('ref_axis',(-1.75746881493119E-17,0.866025403784434,-0.500000000000009));
#22666=DIRECTION('',(0.,-0.866025403784434,0.500000000000009));
#22667=DIRECTION('',(-0.994132040497618,-0.0764901498757908,-0.07649014987579));
#22668=DIRECTION('center_axis',(0.104528463267654,-0.861281226008775,-0.497260947684136));
#22669=DIRECTION('ref_axis',(8.84532624015479E-17,0.499999999999999,-0.866025403784439));
#22670=DIRECTION('',(0.,-0.5,0.866025403784439));
#22671=DIRECTION('',(-0.993634572314886,-0.111560032084303,-0.0156427600493608));
#22672=DIRECTION('center_axis',(0.104528463267654,-0.96482795802185,0.241206989505466));
#22673=DIRECTION('ref_axis',(3.16327731693601E-17,-0.242535625036336,-0.970142500145331));
#22674=DIRECTION('',(0.,0.242535625036336,0.970142500145331));
#22675=DIRECTION('',(-0.985727427293419,-0.132693722013437,-0.103604127426077));
#22676=DIRECTION('center_axis',(0.104528463267654,-3.63204311424904E-15,
-0.994521895368273));
#22677=DIRECTION('ref_axis',(-0.994521895368273,-6.31025267670437E-32,-0.104528463267654));
#22678=DIRECTION('',(0.,-1.,3.65204942310906E-15));
#22679=DIRECTION('',(-0.985727427293419,0.132693722013436,-0.103604127426078));
#22680=DIRECTION('center_axis',(0.104528463267654,0.964827958021852,0.241206989505459));
#22681=DIRECTION('ref_axis',(-2.43308567694987E-17,-0.242535625036329,0.970142500145333));
#22682=DIRECTION('',(0.,0.242535625036329,-0.970142500145333));
#22683=DIRECTION('',(-0.993634572314886,0.111560032084303,-0.0156427600493608));
#22684=DIRECTION('center_axis',(0.104528463267654,0.861281226008778,-0.49726094768413));
#22685=DIRECTION('ref_axis',(5.38148870333637E-17,0.499999999999993,0.866025403784443));
#22686=DIRECTION('',(0.,-0.499999999999993,-0.866025403784443));
#22687=DIRECTION('',(-0.994132040497618,0.0764901498757906,-0.0764901498757907));
#22688=DIRECTION('center_axis',(0.104528463267654,0.497260947684129,-0.861281226008779));
#22689=DIRECTION('ref_axis',(2.61266480593264E-18,0.866025403784443,0.499999999999992));
#22690=DIRECTION('',(0.,-0.866025403784443,-0.499999999999992));
#22691=DIRECTION('center_axis',(-1.,0.,0.));
#22692=DIRECTION('ref_axis',(0.,0.,1.));
#22693=DIRECTION('center_axis',(-1.,0.,0.));
#22694=DIRECTION('ref_axis',(0.,0.,1.));
#22695=DIRECTION('center_axis',(0.,1.,-1.22464679914735E-16));
#22696=DIRECTION('ref_axis',(0.,-1.22464679914735E-16,-1.));
#48581=CARTESIAN_POINT('',(0.,0.,0.));
#48582=CARTESIAN_POINT('Origin',(0.0016,0.,0.));
#48583=CARTESIAN_POINT('',(-0.00145274996309991,0.000934523397478773,-0.000217677932639515));
#48584=CARTESIAN_POINT('',(-0.00154602165644221,0.000569150220513997,-0.000136439597205102));
#48585=CARTESIAN_POINT('Origin',(0.00156503616117409,8.06815870157537E-5,
0.000322726348063015));
#48586=CARTESIAN_POINT('',(-0.00145274996309991,0.000934523397478773,0.000217677932639515));
#48587=CARTESIAN_POINT('Origin',(0.00166379421431252,0.000606961405040141,
0.));
#48588=CARTESIAN_POINT('',(-0.00154602165644221,0.000569150220513997,0.000136439597205102));
#48589=CARTESIAN_POINT('Origin',(0.00156503616117409,8.06815870157537E-5,
-0.000322726348063015));
#48590=CARTESIAN_POINT('',(-0.00157234339721419,0.000296847915734235,0.000296847915734239));
#48591=CARTESIAN_POINT('Origin',(0.00160749262454254,3.56437803082174E-5,
6.17368384676569E-5));
#48592=CARTESIAN_POINT('',(-0.00154602165644221,0.000136439597205108,0.000569150220513995));
#48593=CARTESIAN_POINT('Origin',(0.00160749262454254,6.17368384676549E-5,
3.56437803082147E-5));
#48594=CARTESIAN_POINT('',(-0.00145274996309991,0.000217677932639525,0.000934523397478771));
#48595=CARTESIAN_POINT('Origin',(0.00156503616117409,-0.000322726348063014,
8.06815870157571E-5));
#48596=CARTESIAN_POINT('',(-0.00145274996309991,-0.000217677932639505,0.000934523397478775));
#48597=CARTESIAN_POINT('Origin',(0.00166379421431252,6.37287751623816E-18,
0.000606961405040141));
#48598=CARTESIAN_POINT('',(-0.00154602165644221,-0.000136439597205096,0.000569150220513998));
#48599=CARTESIAN_POINT('Origin',(0.00156503616117409,0.000322726348063016,
8.06815870157503E-5));
#48600=CARTESIAN_POINT('',(-0.00157234339721419,-0.000296847915734233,0.000296847915734241));
#48601=CARTESIAN_POINT('Origin',(0.00160749262454254,-6.17368384676559E-5,
3.56437803082175E-5));
#48602=CARTESIAN_POINT('',(-0.00154602165644221,-0.000569150220513996,0.000136439597205106));
#48603=CARTESIAN_POINT('Origin',(0.00160749262454254,-3.5643780308217E-5,
6.17368384676573E-5));
#48604=CARTESIAN_POINT('',(-0.00145274996309991,-0.000934523397478772,0.000217677932639521));
#48605=CARTESIAN_POINT('Origin',(0.00156503616117409,-8.06815870157559E-5,
-0.000322726348063014));
#48606=CARTESIAN_POINT('',(-0.00146025981347714,-0.000935312714559631,1.14542772208728E-19));
#48607=CARTESIAN_POINT('Origin',(0.00166379421431252,-0.000606961405040141,
4.15622446711184E-18));
#48608=CARTESIAN_POINT('',(-0.00089799919935936,-0.002,2.44929359829471E-19));
#48609=CARTESIAN_POINT('Origin',(0.0016,0.,0.));
#48610=CARTESIAN_POINT('',(-0.00089799919935936,-2.44929359829471E-19,-0.002));
#48611=CARTESIAN_POINT('Origin',(-0.00089799919935936,0.,0.));
#48612=CARTESIAN_POINT('Origin',(-0.00089799919935936,0.,0.));
#48613=CARTESIAN_POINT('',(-0.00145274996309991,-0.000934523397478775,-0.000217677932639508));
#48614=CARTESIAN_POINT('Origin',(0.00166379421431252,-0.000606961405040141,
4.15622446711184E-18));
#48615=CARTESIAN_POINT('',(-0.00154602165644221,-0.000569150220513998,-0.000136439597205098));
#48616=CARTESIAN_POINT('Origin',(0.00156503616117409,-8.06815870157514E-5,
0.000322726348063015));
#48617=CARTESIAN_POINT('',(-0.00157234339721419,-0.000296847915734242,-0.000296847915734239));
#48618=CARTESIAN_POINT('Origin',(0.00160749262454254,-3.56437803082212E-5,
-6.17368384676608E-5));
#48619=CARTESIAN_POINT('',(-0.00154602165644221,-0.000136439597205104,-0.000569150220513996));
#48620=CARTESIAN_POINT('Origin',(0.00160749262454254,-6.17368384676611E-5,
-3.56437803082205E-5));
#48621=CARTESIAN_POINT('',(-0.00145274996309991,-0.000217677932639518,-0.000934523397478772));
#48622=CARTESIAN_POINT('Origin',(0.00156503616117409,0.000322726348063015,
-8.06815870157548E-5));
#48623=CARTESIAN_POINT('',(-0.00145274996309991,0.000217677932639511,-0.000934523397478774));
#48624=CARTESIAN_POINT('Origin',(0.00166379421431252,-2.21665304912631E-18,
-0.000606961405040141));
#48625=CARTESIAN_POINT('',(-0.00154602165644221,0.0001364395972051,-0.000569150220513997));
#48626=CARTESIAN_POINT('Origin',(0.00156503616117409,-0.000322726348063015,
-8.06815870157525E-5));
#48627=CARTESIAN_POINT('',(-0.00157234339721419,0.000296847915734235,-0.000296847915734239));
#48628=CARTESIAN_POINT('Origin',(0.00160749262454254,6.17368384676561E-5,
-3.5643780308217E-5));
#48629=CARTESIAN_POINT('Origin',(0.00160749262454254,3.56437803082175E-5,
-6.1736838467657E-5));
#48630=CARTESIAN_POINT('Origin',(0.,0.001,0.));
#48631=CARTESIAN_POINT('',(0.,-2.44929359829471E-19,-0.002));
#48632=CARTESIAN_POINT('Origin',(0.,0.,0.));
#48633=CARTESIAN_POINT('',(0.,-1.34711147906209E-19,-0.0011));
#48634=CARTESIAN_POINT('Origin',(0.,0.,0.));
#48635=CARTESIAN_POINT('Origin',(0.,0.,0.));
#48636=CARTESIAN_POINT('',(0.,-2.44929359829471E-19,-0.002));
#48637=CARTESIAN_POINT('Origin',(0.0045,0.001,0.));
#48638=CARTESIAN_POINT('',(0.0045,-9.79717439317885E-20,-0.000800000000000002));
#48639=CARTESIAN_POINT('Origin',(0.0045,0.,0.));
#48640=CARTESIAN_POINT('Origin',(0.,0.,0.));
#48641=CARTESIAN_POINT('',(0.0001,-1.22464679914735E-19,-0.001));
#48642=CARTESIAN_POINT('Origin',(0.0001,0.,0.));
#48643=CARTESIAN_POINT('',(0.00415358983848623,-1.22464679914735E-19,-0.001));
#48644=CARTESIAN_POINT('',(0.,-1.22464679914735E-19,-0.001));
#48645=CARTESIAN_POINT('Origin',(0.00415358983848623,0.,0.));
#48646=CARTESIAN_POINT('Origin',(0.00415358983848623,0.,0.));
#48647=CARTESIAN_POINT('',(0.00415358983848623,-1.22464679914735E-19,-0.001));
#48648=CARTESIAN_POINT('Origin',(-0.0016,0.00095,-0.0002375));
#48649=CARTESIAN_POINT('',(-0.00075,0.000556618474827239,-4.70664976705276E-5));
#48650=CARTESIAN_POINT('',(-0.0016,0.00057,-0.0001425));
#48651=CARTESIAN_POINT('',(-0.00075,0.000860661400024175,-0.000123077228969761));
#48652=CARTESIAN_POINT('',(-0.00075,2.16677931850071E-5,8.66711727400304E-5));
#48653=CARTESIAN_POINT('',(-0.00153787007542131,0.000943469881790042,-0.000229136378665655));
#48654=CARTESIAN_POINT('Origin',(-0.0016,0.00095,0.0002375));
#48655=CARTESIAN_POINT('',(-0.00075,0.000860661400024175,0.000123077228969761));
#48656=CARTESIAN_POINT('',(-0.00075,0.000860661400024175,-4.33680868994202E-19));
#48657=CARTESIAN_POINT('',(-0.0016,0.00095,0.0002375));
#48658=CARTESIAN_POINT('Origin',(-0.0016,0.00095,0.0002375));
#48659=CARTESIAN_POINT('',(-0.00075,0.000556618474827239,4.70664976705276E-5));
#48660=CARTESIAN_POINT('',(-0.00075,2.16677931850068E-5,-8.66711727400304E-5));
#48661=CARTESIAN_POINT('',(-0.00161643715208567,0.00057025876960518,0.00014434547646101));
#48662=CARTESIAN_POINT('Origin',(-0.0016,0.00057,0.0001425));
#48663=CARTESIAN_POINT('',(-0.00075,0.000233575465858467,0.000233575465858471));
#48664=CARTESIAN_POINT('',(-0.00075,0.000159535010031724,0.000276322742960963));
#48665=CARTESIAN_POINT('',(-0.00160871040111109,0.000299646052667046,0.000299646052667049));
#48666=CARTESIAN_POINT('Origin',(-0.0016,0.000142500000000006,0.00057));
#48667=CARTESIAN_POINT('',(-0.00075,4.70664976705335E-5,0.000556618474827239));
#48668=CARTESIAN_POINT('',(-0.00075,0.000276322742960963,0.000159535010031717));
#48669=CARTESIAN_POINT('',(-0.0016,0.000142500000000006,0.00057));
#48670=CARTESIAN_POINT('Origin',(-0.0016,0.0002375,0.00095));
#48671=CARTESIAN_POINT('',(-0.00075,0.00012307722896977,0.000860661400024173));
#48672=CARTESIAN_POINT('',(-0.00075,-8.66711727400301E-5,2.16677931850079E-5));
#48673=CARTESIAN_POINT('',(-0.00153787007542131,0.000229136378665665,0.00094346988179004));
#48674=CARTESIAN_POINT('Origin',(-0.0016,-0.00023749999999999,0.00095));
#48675=CARTESIAN_POINT('',(-0.00075,-0.000123077228969752,0.000860661400024176));
#48676=CARTESIAN_POINT('',(-0.00075,8.44032546730324E-18,0.000860661400024174));
#48677=CARTESIAN_POINT('',(-0.0016,-0.00023749999999999,0.00095));
#48678=CARTESIAN_POINT('Origin',(-0.0016,-0.00023749999999999,0.00095));
#48679=CARTESIAN_POINT('',(-0.00075,-4.70664976705218E-5,0.00055661847482724));
#48680=CARTESIAN_POINT('',(-0.00075,8.66711727400305E-5,2.16677931850063E-5));
#48681=CARTESIAN_POINT('',(-0.00161643715208567,-0.000144345476461004,0.000570258769605181));
#48682=CARTESIAN_POINT('Origin',(-0.0016,-0.000142499999999994,0.00057));
#48683=CARTESIAN_POINT('',(-0.00075,-0.000233575465858466,0.000233575465858473));
#48684=CARTESIAN_POINT('',(-0.00075,-0.000276322742960961,0.000159535010031725));
#48685=CARTESIAN_POINT('',(-0.00160871040111109,-0.000299646052667044,0.000299646052667051));
#48686=CARTESIAN_POINT('Origin',(-0.0016,-0.00057,0.000142500000000004));
#48687=CARTESIAN_POINT('',(-0.00075,-0.000556618474827239,4.70664976705315E-5));
#48688=CARTESIAN_POINT('',(-0.00075,-0.000159535010031723,0.000276322742960963));
#48689=CARTESIAN_POINT('',(-0.0016,-0.00057,0.000142500000000004));
#48690=CARTESIAN_POINT('Origin',(-0.0016,-0.00095,0.000237500000000007));
#48691=CARTESIAN_POINT('',(-0.00075,-0.000860661400024174,0.000123077228969767));
#48692=CARTESIAN_POINT('',(-0.00075,-2.16677931850086E-5,-8.667117274003E-5));
#48693=CARTESIAN_POINT('',(-0.00153787007542131,-0.000943469881790041,0.000229136378665661));
#48694=CARTESIAN_POINT('Origin',(-0.0016,-0.00095,-0.000237499999999993));
#48695=CARTESIAN_POINT('',(-0.00075,-0.000860661400024175,-0.000123077228969755));
#48696=CARTESIAN_POINT('',(-0.00075,-0.000860661400024175,5.45977782372553E-18));
#48697=CARTESIAN_POINT('',(-0.0016,-0.00095,-0.000237499999999993));
#48698=CARTESIAN_POINT('Origin',(-0.0016,-0.00095,-0.000237499999999993));
#48699=CARTESIAN_POINT('',(-0.00075,-0.000556618474827239,-4.70664976705236E-5));
#48700=CARTESIAN_POINT('',(-0.00075,-2.16677931850076E-5,8.66711727400303E-5));
#48701=CARTESIAN_POINT('',(-0.00161643715208567,-0.000570258769605181,-0.000144345476461006));
#48702=CARTESIAN_POINT('Origin',(-0.0016,-0.00057,-0.000142499999999996));
#48703=CARTESIAN_POINT('',(-0.00075,-0.000233575465858474,-0.000233575465858472));
#48704=CARTESIAN_POINT('',(-0.00075,-0.000159535010031733,-0.000276322742960964));
#48705=CARTESIAN_POINT('',(-0.00160871040111109,-0.000299646052667053,-0.000299646052667049));
#48706=CARTESIAN_POINT('Origin',(-0.0016,-0.000142500000000002,-0.00057));
#48707=CARTESIAN_POINT('',(-0.00075,-4.70664976705294E-5,-0.000556618474827239));
#48708=CARTESIAN_POINT('',(-0.00075,-0.000276322742960965,-0.000159535010031729));
#48709=CARTESIAN_POINT('',(-0.0016,-0.000142500000000002,-0.00057));
#48710=CARTESIAN_POINT('Origin',(-0.0016,-0.000237500000000003,-0.00095));
#48711=CARTESIAN_POINT('',(-0.00075,-0.000123077228969764,-0.000860661400024174));
#48712=CARTESIAN_POINT('',(-0.00075,8.667117274003E-5,-2.16677931850084E-5));
#48713=CARTESIAN_POINT('',(-0.00153787007542131,-0.000229136378665658,-0.000943469881790042));
#48714=CARTESIAN_POINT('Origin',(-0.0016,0.000237499999999997,-0.00095));
#48715=CARTESIAN_POINT('',(-0.00075,0.000123077228969758,-0.000860661400024175));
#48716=CARTESIAN_POINT('',(-0.00075,-3.73948916431755E-18,-0.000860661400024175));
#48717=CARTESIAN_POINT('',(-0.0016,0.000237499999999997,-0.00095));
#48718=CARTESIAN_POINT('Origin',(-0.0016,0.000237499999999997,-0.00095));
#48719=CARTESIAN_POINT('',(-0.00075,4.70664976705257E-5,-0.00055661847482724));
#48720=CARTESIAN_POINT('',(-0.00075,-8.66711727400302E-5,-2.16677931850075E-5));
#48721=CARTESIAN_POINT('',(-0.00161643715208567,0.000144345476461008,-0.00057025876960518));
#48722=CARTESIAN_POINT('Origin',(-0.0016,0.000142499999999998,-0.00057));
#48723=CARTESIAN_POINT('',(-0.00075,0.000233575465858468,-0.000233575465858471));
#48724=CARTESIAN_POINT('',(-0.00075,0.000276322742960961,-0.000159535010031724));
#48725=CARTESIAN_POINT('',(-0.00160871040111109,0.000299646052667046,-0.000299646052667049));
#48726=CARTESIAN_POINT('Origin',(-0.0016,0.00057,-0.0001425));
#48727=CARTESIAN_POINT('',(-0.00075,0.000159535010031724,-0.000276322742960963));
#48728=CARTESIAN_POINT('Origin',(-0.00075,-5.96311194867027E-19,-4.33680868994202E-19));
#48729=CARTESIAN_POINT('Origin',(0.0001,0.,0.));
#48730=CARTESIAN_POINT('Origin',(0.0001,-1.34711147906209E-19,-0.0011));
#54559=UNCERTAINTY_MEASURE_WITH_UNIT(LENGTH_MEASURE(1.E-5),#54581,
'DISTANCE_ACCURACY_VALUE',
'Maximum model space distance between geometric entities at asserted c
onnectivities');
#54564=UNCERTAINTY_MEASURE_WITH_UNIT(LENGTH_MEASURE(1.E-5),#54581,
'DISTANCE_ACCURACY_VALUE',
'Maximum model space distance between geometric entities at asserted c
onnectivities');
#54575=(
GEOMETRIC_REPRESENTATION_CONTEXT(3)
GLOBAL_UNCERTAINTY_ASSIGNED_CONTEXT((#54559))
GLOBAL_UNIT_ASSIGNED_CONTEXT((#54581,#54582,#54583))
REPRESENTATION_CONTEXT('','3D')
);
#54580=(
GEOMETRIC_REPRESENTATION_CONTEXT(3)
GLOBAL_UNCERTAINTY_ASSIGNED_CONTEXT((#54564))
GLOBAL_UNIT_ASSIGNED_CONTEXT((#54581,#54582,#54583))
REPRESENTATION_CONTEXT('','3D')
);
#54581=(
LENGTH_UNIT()
NAMED_UNIT(*)
SI_UNIT($,.METRE.)
);
#54582=(
NAMED_UNIT(*)
PLANE_ANGLE_UNIT()
SI_UNIT($,.RADIAN.)
);
#54583=(
NAMED_UNIT(*)
SI_UNIT($,.STERADIAN.)
SOLID_ANGLE_UNIT()
);
#54594=SHAPE_DEFINITION_REPRESENTATION(#54609,#54639);
#54609=PRODUCT_DEFINITION_SHAPE('',$,#54655);
#54639=SHAPE_REPRESENTATION('',(#19079),#54575);
#54644=PRODUCT_DEFINITION_CONTEXT('part definition',#54691,'design');
#54655=PRODUCT_DEFINITION('Part_3','Part_3',#54670,#54644);
#54670=PRODUCT_DEFINITION_FORMATION('',$,#54703);
#54691=APPLICATION_CONTEXT(
'Core Data for Automotive Mechanical Design Process');
#54692=PRODUCT_CONTEXT('part definition',#54691,'mechanical');
#54703=PRODUCT('Part_3','Part_3','Part 1',(#54692));
#54716=PRESENTATION_STYLE_ASSIGNMENT((#54726));
#54726=SURFACE_STYLE_USAGE(.BOTH.,#54736);
#54736=SURFACE_SIDE_STYLE('',(#54746));
#54746=SURFACE_STYLE_FILL_AREA(#54756);
#54756=FILL_AREA_STYLE('Opaque(76,76,76)',(#54766));
#54766=FILL_AREA_STYLE_COLOUR('Opaque(76,76,76)',#54776);
#54776=COLOUR_RGB('Opaque(76,76,76)', 0.08235294, 0.09019608, 0.10196078);
ENDSEC;
END-ISO-10303-21;
